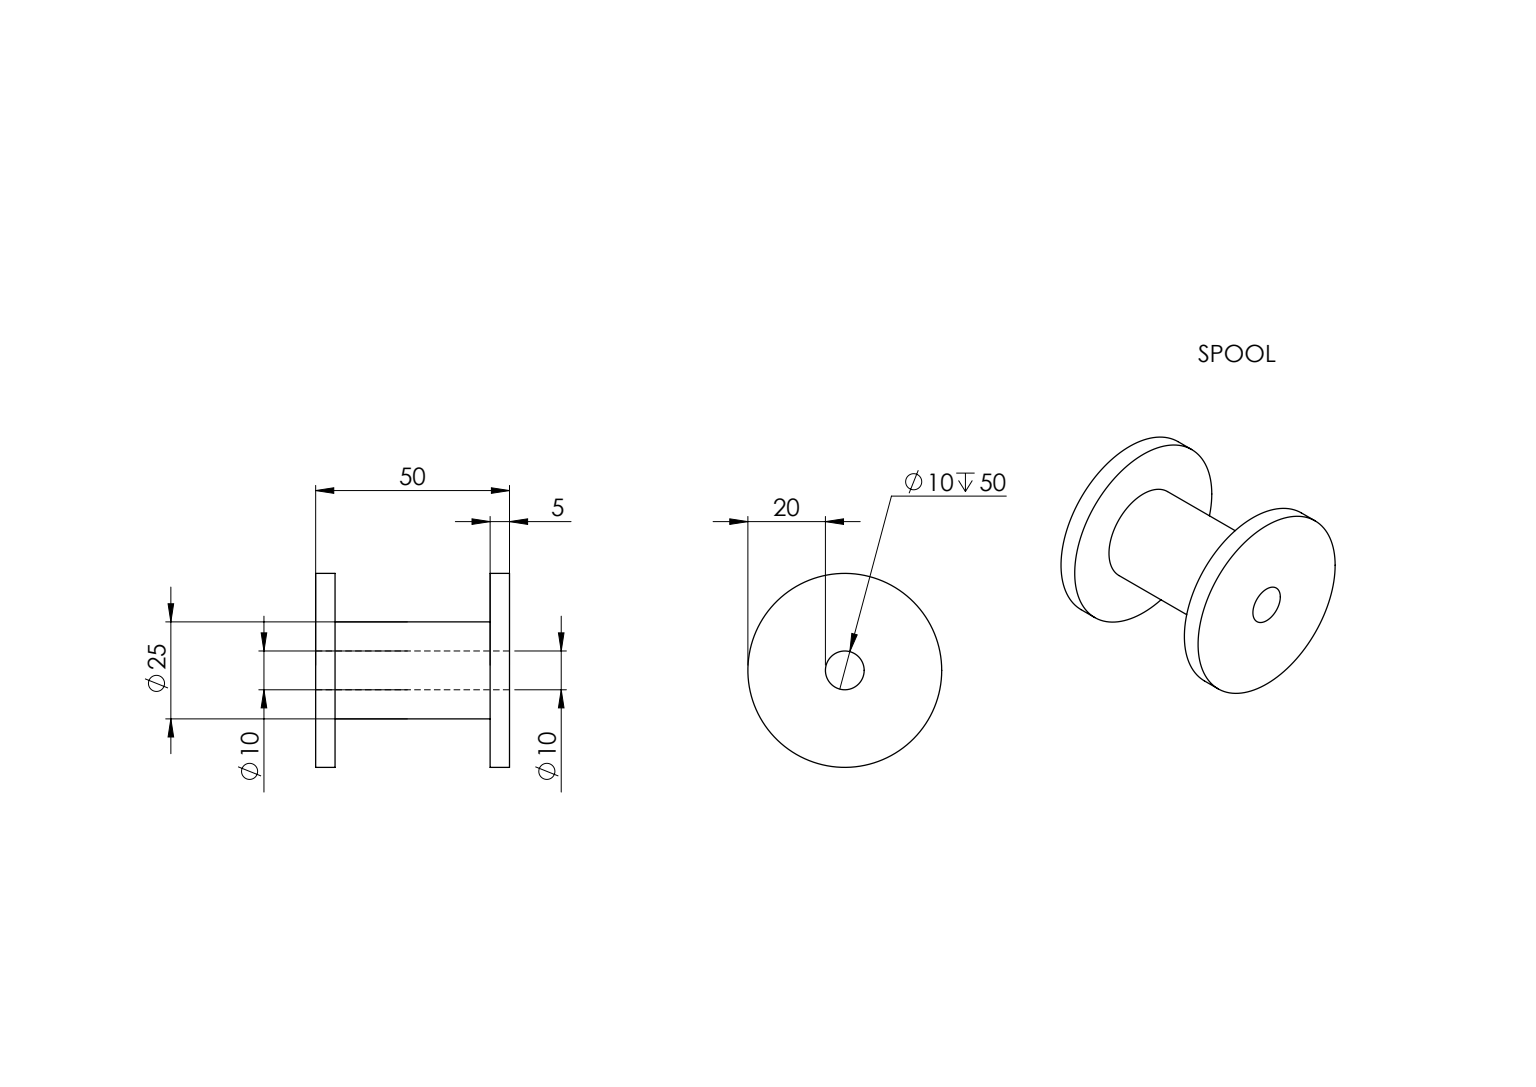
ISO-10303-21;
HEADER;
FILE_DESCRIPTION (('STEP AP214'),
    '1' );
FILE_NAME ('spool.step',
    '2026-10-27T08:02:39',
    ( '' ),
    ( '' ),
    'SwSTEP 2.0',
    'SolidWorks 2026',
    '' );
FILE_SCHEMA (( 'AUTOMOTIVE_DESIGN' ));
ENDSEC;

DATA;
#97=( NAMED_UNIT ( * ) SI_UNIT ( $, .STERADIAN. ) SOLID_ANGLE_UNIT ( ) );
#142=FACE_BOUND ( 'NONE', #771, .T. ) ;
#196=DIRECTION ( 'NONE',  ( 0.000000000000000000, 0.000000000000000000, 1.000000000000000000 ) ) ;
#212=CARTESIAN_POINT ( 'NONE',  ( 0.000000000000000000, 0.000000000000000000, 0.000000000000000000 ) ) ;
#226=DIRECTION ( 'NONE',  ( 1.000000000000000000, 0.000000000000000000, 0.000000000000000000 ) ) ;
#270=CARTESIAN_POINT ( 'NONE',  ( 25.00000000000000000, 0.000000000000000000, 0.000000000000000000 ) ) ;
#326=LINE ( 'NONE', #5141, #3967 ) ;
#355=LINE ( 'NONE', #8000, #10056 ) ;
#393=DIRECTION ( 'NONE',  ( 1.000000000000000000, 0.000000000000000000, 0.000000000000000000 ) ) ;
#459=CIRCLE ( 'NONE', #3072, 12.50000000000000000 ) ;
#620=AXIS2_PLACEMENT_3D ( 'NONE', #9988, #3488, #10977 ) ;
#625=CARTESIAN_POINT ( 'NONE',  ( -25.00000000000000000, 0.000000000000000000, 0.000000000000000000 ) ) ;
#642=CIRCLE ( 'NONE', #6043, 25.00000000000000000 ) ;
#671=FACE_BOUND ( 'NONE', #6645, .T. ) ;
#771=EDGE_LOOP ( 'NONE', ( #6888, #1800 ) ) ;
#957=DIRECTION ( 'NONE',  ( 1.000000000000000000, 0.000000000000000000, 0.000000000000000000 ) ) ;
#961=SURFACE_SIDE_STYLE ('',( #5858 ) ) ;
#980=EDGE_CURVE ( 'NONE', #1358, #1101, #4200, .T. ) ;
#1046=CARTESIAN_POINT ( 'NONE',  ( 20.00000000000000000, 3.061616997868383043E-15, 25.00000000000000000 ) ) ;
#1054=DIRECTION ( 'NONE',  ( 1.000000000000000000, 0.000000000000000000, 0.000000000000000000 ) ) ;
#1071=DIRECTION ( 'NONE',  ( 0.000000000000000000, 0.000000000000000000, 1.000000000000000000 ) ) ;
#1097=( NAMED_UNIT ( * ) PLANE_ANGLE_UNIT ( ) SI_UNIT ( $, .RADIAN. ) );
#1101=VERTEX_POINT ( 'NONE', #1046 ) ;
#1135=CARTESIAN_POINT ( 'NONE',  ( 25.00000000000000000, 0.000000000000000000, 0.000000000000000000 ) ) ;
#1142=FACE_OUTER_BOUND ( 'NONE', #11815, .T. ) ;
#1171=EDGE_CURVE ( 'NONE', #6684, #6331, #3612, .T. ) ;
#1213=FILL_AREA_STYLE ('',( #6917 ) ) ;
#1214=ORIENTED_EDGE ( 'NONE', *, *, #7345, .F. ) ;
#1267=ORIENTED_EDGE ( 'NONE', *, *, #10956, .F. ) ;
#1301=ORIENTED_EDGE ( 'NONE', *, *, #2405, .T. ) ;
#1314=FACE_OUTER_BOUND ( 'NONE', #4071, .T. ) ;
#1327=DIRECTION ( 'NONE',  ( 0.000000000000000000, 0.000000000000000000, -1.000000000000000000 ) ) ;
#1349=ORIENTED_EDGE ( 'NONE', *, *, #3855, .T. ) ;
#1358=VERTEX_POINT ( 'NONE', #5530 ) ;
#1364=VECTOR ( 'NONE', #12094, 1000.000000000000000 ) ;
#1402=CARTESIAN_POINT ( 'NONE',  ( 25.00000000000000000, 0.000000000000000000, 0.000000000000000000 ) ) ;
#1412=ORIENTED_EDGE ( 'NONE', *, *, #980, .F. ) ;
#1470=CARTESIAN_POINT ( 'NONE',  ( -20.00000000000000000, 0.000000000000000000, 0.000000000000000000 ) ) ;
#1514=DIRECTION ( 'NONE',  ( 0.000000000000000000, 0.000000000000000000, -1.000000000000000000 ) ) ;
#1630=DIRECTION ( 'NONE',  ( 1.000000000000000000, 0.000000000000000000, 0.000000000000000000 ) ) ;
#1657=VERTEX_POINT ( 'NONE', #3156 ) ;
#1730=DIRECTION ( 'NONE',  ( 0.000000000000000000, 0.000000000000000000, -1.000000000000000000 ) ) ;
#1731=EDGE_CURVE ( 'NONE', #6756, #7499, #326, .T. ) ;
#1747=VERTEX_POINT ( 'NONE', #10142 ) ;
#1777=CARTESIAN_POINT ( 'NONE',  ( -25.00000000000000000, 6.123233995736766282E-16, -5.000000000000000000 ) ) ;
#1793=ORIENTED_EDGE ( 'NONE', *, *, #9745, .F. ) ;
#1795=LINE ( 'NONE', #4305, #6226 ) ;
#1800=ORIENTED_EDGE ( 'NONE', *, *, #4057, .T. ) ;
#1916=EDGE_LOOP ( 'NONE', ( #11600, #6853 ) ) ;
#1917=( LENGTH_UNIT ( ) NAMED_UNIT ( * ) SI_UNIT ( .MILLI., .METRE. ) );
#1988=CARTESIAN_POINT ( 'NONE',  ( 25.00000000000000000, 0.000000000000000000, 0.000000000000000000 ) ) ;
#2080=MECHANICAL_DESIGN_GEOMETRIC_PRESENTATION_REPRESENTATION('',(#3887),#10866);
#2081=DIRECTION ( 'NONE',  ( 1.000000000000000000, -0.000000000000000000, -0.000000000000000000 ) ) ;
#2083=ORIENTED_EDGE ( 'NONE', *, *, #7345, .T. ) ;
#2120=ORIENTED_EDGE ( 'NONE', *, *, #9829, .F. ) ;
#2122=CARTESIAN_POINT ( 'NONE',  ( -19.99999999999999645, 0.000000000000000000, 12.50000000000000000 ) ) ;
#2150=SHAPE_DEFINITION_REPRESENTATION ( #8046, #7217 ) ;
#2179=ADVANCED_FACE ( 'NONE', ( #8194, #3447 ), #9138, .T. ) ;
#2211=ORIENTED_EDGE ( 'NONE', *, *, #8931, .F. ) ;
#2280=DIRECTION ( 'NONE',  ( 0.000000000000000000, 0.000000000000000000, -1.000000000000000000 ) ) ;
#2288=AXIS2_PLACEMENT_3D ( 'NONE', #7775, #11643, #9901 ) ;
#2395=( LENGTH_UNIT ( ) NAMED_UNIT ( * ) SI_UNIT ( .MILLI., .METRE. ) );
#2405=EDGE_CURVE ( 'NONE', #12064, #3807, #9823, .T. ) ;
#2527=DIRECTION ( 'NONE',  ( 1.000000000000000000, 0.000000000000000000, 0.000000000000000000 ) ) ;
#2578=ORIENTED_EDGE ( 'NONE', *, *, #10956, .T. ) ;
#2623=VERTEX_POINT ( 'NONE', #1777 ) ;
#2628=EDGE_CURVE ( 'NONE', #6331, #6684, #11193, .T. ) ;
#2679=EDGE_CURVE ( 'NONE', #6067, #9683, #10623, .T. ) ;
#2791=DIRECTION ( 'NONE',  ( -1.000000000000000000, -0.000000000000000000, -0.000000000000000000 ) ) ;
#2915=LINE ( 'NONE', #9730, #10436 ) ;
#2988=CLOSED_SHELL ( 'NONE', ( #5813, #5217, #3491, #8176, #5004, #4607, #4938, #11804, #6014, #11882, #2179, #7611 ) ) ;
#3002=FACE_OUTER_BOUND ( 'NONE', #7243, .T. ) ;
#3072=AXIS2_PLACEMENT_3D ( 'NONE', #4632, #4174, #7889 ) ;
#3078=ORIENTED_EDGE ( 'NONE', *, *, #11451, .T. ) ;
#3081=FACE_OUTER_BOUND ( 'NONE', #4296, .T. ) ;
#3090=CYLINDRICAL_SURFACE ( 'NONE', #11035, 5.000000000000000000 ) ;
#3156=CARTESIAN_POINT ( 'NONE',  ( -19.99999999999999645, 1.530808498934191521E-15, -12.50000000000000000 ) ) ;
#3211=ORIENTED_EDGE ( 'NONE', *, *, #12328, .F. ) ;
#3291=EDGE_LOOP ( 'NONE', ( #5014, #12285, #7753, #4819 ) ) ;
#3379=DIRECTION ( 'NONE',  ( 0.000000000000000000, 0.000000000000000000, -1.000000000000000000 ) ) ;
#3447=FACE_BOUND ( 'NONE', #1916, .T. ) ;
#3488=DIRECTION ( 'NONE',  ( 1.000000000000000000, 0.000000000000000000, 0.000000000000000000 ) ) ;
#3491=ADVANCED_FACE ( 'NONE', ( #1314 ), #3090, .F. ) ;
#3563=ORIENTED_EDGE ( 'NONE', *, *, #4057, .F. ) ;
#3574=CIRCLE ( 'NONE', #5763, 25.00000000000000000 ) ;
#3598=DIRECTION ( 'NONE',  ( 0.000000000000000000, 0.000000000000000000, -1.000000000000000000 ) ) ;
#3612=CIRCLE ( 'NONE', #6408, 25.00000000000000000 ) ;
#3635=CARTESIAN_POINT ( 'NONE',  ( 20.00000000000000000, 0.000000000000000000, 0.000000000000000000 ) ) ;
#3807=VERTEX_POINT ( 'NONE', #9382 ) ;
#3852=PRESENTATION_STYLE_ASSIGNMENT (( #5032 ) ) ;
#3855=EDGE_CURVE ( 'NONE', #9683, #6067, #459, .T. ) ;
#3859=COLOUR_RGB ( '',0.8941176470588234615, 0.8941176470588234615, 0.8941176470588234615 ) ;
#3869=CIRCLE ( 'NONE', #7870, 5.000000000000000000 ) ;
#3871=VERTEX_POINT ( 'NONE', #2122 ) ;
#3873=EDGE_CURVE ( 'NONE', #12064, #8607, #355, .T. ) ;
#3887=STYLED_ITEM('',(#12412),#4645);
#3905=UNCERTAINTY_MEASURE_WITH_UNIT (LENGTH_MEASURE( 1.000000000000000082E-05 ), #1917, 'distance_accuracy_value', 'NONE');
#3910=CARTESIAN_POINT ( 'NONE',  ( 25.00000000000000000, 6.123233995736766282E-16, -5.000000000000000000 ) ) ;
#3949=CARTESIAN_POINT ( 'NONE',  ( -19.99999999999999645, 0.000000000000000000, 0.000000000000000000 ) ) ;
#3956=FACE_OUTER_BOUND ( 'NONE', #11536, .T. ) ;
#3967=VECTOR ( 'NONE', #5024, 1000.000000000000000 ) ;
#3973=EDGE_CURVE ( 'NONE', #3871, #1657, #8067, .T. ) ;
#3980=ORIENTED_EDGE ( 'NONE', *, *, #9518, .T. ) ;
#4031=VECTOR ( 'NONE', #4905, 1000.000000000000000 ) ;
#4032=CIRCLE ( 'NONE', #9832, 25.00000000000000000 ) ;
#4035=DIRECTION ( 'NONE',  ( 0.000000000000000000, 0.000000000000000000, 1.000000000000000000 ) ) ;
#4038=CARTESIAN_POINT ( 'NONE',  ( 25.00000000000000000, 0.000000000000000000, 0.000000000000000000 ) ) ;
#4057=EDGE_CURVE ( 'NONE', #2623, #7499, #3869, .T. ) ;
#4071=EDGE_LOOP ( 'NONE', ( #3980, #9462, #7743, #9623 ) ) ;
#4083=DIRECTION ( 'NONE',  ( -1.000000000000000000, -0.000000000000000000, -0.000000000000000000 ) ) ;
#4093=AXIS2_PLACEMENT_3D ( 'NONE', #3635, #6273, #1514 ) ;
#4104=FACE_OUTER_BOUND ( 'NONE', #3291, .T. ) ;
#4111=ORIENTED_EDGE ( 'NONE', *, *, #9518, .F. ) ;
#4132=DIRECTION ( 'NONE',  ( -1.000000000000000000, -0.000000000000000000, -0.000000000000000000 ) ) ;
#4152=CARTESIAN_POINT ( 'NONE',  ( 25.00000000000000000, 0.000000000000000000, 0.000000000000000000 ) ) ;
#4174=DIRECTION ( 'NONE',  ( 1.000000000000000000, 0.000000000000000000, 0.000000000000000000 ) ) ;
#4200=CIRCLE ( 'NONE', #10797, 25.00000000000000000 ) ;
#4266=AXIS2_PLACEMENT_3D ( 'NONE', #4038, #393, #2280 ) ;
#4296=EDGE_LOOP ( 'NONE', ( #2120, #2578, #7552, #3563 ) ) ;
#4305=CARTESIAN_POINT ( 'NONE',  ( 25.00000000000000000, 1.530808498934191521E-15, -12.50000000000000000 ) ) ;
#4325=CARTESIAN_POINT ( 'NONE',  ( 20.00000000000000000, 1.530808498934191521E-15, -12.50000000000000000 ) ) ;
#4337=CYLINDRICAL_SURFACE ( 'NONE', #6991, 12.50000000000000000 ) ;
#4371=DIRECTION ( 'NONE',  ( 1.000000000000000000, -0.000000000000000000, -0.000000000000000000 ) ) ;
#4414=PLANE ( 'NONE',  #620 ) ;
#4421=DIRECTION ( 'NONE',  ( 1.000000000000000000, 0.000000000000000000, 0.000000000000000000 ) ) ;
#4445=DIRECTION ( 'NONE',  ( 0.000000000000000000, 0.000000000000000000, -1.000000000000000000 ) ) ;
#4452=VECTOR ( 'NONE', #7486, 1000.000000000000000 ) ;
#4480=ORIENTED_EDGE ( 'NONE', *, *, #2679, .F. ) ;
#4482=CARTESIAN_POINT ( 'NONE',  ( 20.00000000000000000, 0.000000000000000000, -25.00000000000000000 ) ) ;
#4516=LINE ( 'NONE', #6466, #8844 ) ;
#4552=ORIENTED_EDGE ( 'NONE', *, *, #1171, .T. ) ;
#4574=DIRECTION ( 'NONE',  ( -1.000000000000000000, -0.000000000000000000, -0.000000000000000000 ) ) ;
#4607=ADVANCED_FACE ( 'NONE', ( #6971, #7919 ), #10777, .T. ) ;
#4632=CARTESIAN_POINT ( 'NONE',  ( 20.00000000000000000, 0.000000000000000000, 0.000000000000000000 ) ) ;
#4645=MANIFOLD_SOLID_BREP ( 'Mirror2', #2988 ) ;
#4819=ORIENTED_EDGE ( 'NONE', *, *, #12183, .F. ) ;
#4905=DIRECTION ( 'NONE',  ( -1.000000000000000000, 0.000000000000000000, 0.000000000000000000 ) ) ;
#4938=ADVANCED_FACE ( 'NONE', ( #142, #3956 ), #7528, .F. ) ;
#5004=ADVANCED_FACE ( 'NONE', ( #1142 ), #7143, .T. ) ;
#5014=ORIENTED_EDGE ( 'NONE', *, *, #3855, .F. ) ;
#5024=DIRECTION ( 'NONE',  ( -1.000000000000000000, -0.000000000000000000, -0.000000000000000000 ) ) ;
#5031=AXIS2_PLACEMENT_3D ( 'NONE', #9171, #2527, #3598 ) ;
#5032=SURFACE_STYLE_USAGE ( .BOTH. , #961 ) ;
#5035=PRODUCT_CONTEXT ( 'NONE', #10489, 'mechanical' ) ;
#5084=EDGE_LOOP ( 'NONE', ( #9657, #11921, #6220, #1214 ) ) ;
#5141=CARTESIAN_POINT ( 'NONE',  ( 25.00000000000000000, 0.000000000000000000, 5.000000000000000000 ) ) ;
#5217=ADVANCED_FACE ( 'NONE', ( #9331 ), #11008, .T. ) ;
#5282=DIRECTION ( 'NONE',  ( -1.000000000000000000, 0.000000000000000000, 0.000000000000000000 ) ) ;
#5521=CARTESIAN_POINT ( 'NONE',  ( -25.00000000000000000, 0.000000000000000000, 5.000000000000000000 ) ) ;
#5530=CARTESIAN_POINT ( 'NONE',  ( 20.00000000000000000, 0.000000000000000000, -25.00000000000000000 ) ) ;
#5627=ORIENTED_EDGE ( 'NONE', *, *, #11451, .F. ) ;
#5679=ORIENTED_EDGE ( 'NONE', *, *, #3873, .T. ) ;
#5705=DIRECTION ( 'NONE',  ( 0.000000000000000000, 0.000000000000000000, -1.000000000000000000 ) ) ;
#5716=LINE ( 'NONE', #10587, #4031 ) ;
#5763=AXIS2_PLACEMENT_3D ( 'NONE', #10625, #6884, #10687 ) ;
#5782=( NAMED_UNIT ( * ) PLANE_ANGLE_UNIT ( ) SI_UNIT ( $, .RADIAN. ) );
#5813=ADVANCED_FACE ( 'NONE', ( #5881 ), #5988, .T. ) ;
#5858=SURFACE_STYLE_FILL_AREA ( #1213 ) ;
#5881=FACE_OUTER_BOUND ( 'NONE', #6089, .T. ) ;
#5893=CARTESIAN_POINT ( 'NONE',  ( 25.00000000000000000, 0.000000000000000000, 0.000000000000000000 ) ) ;
#5988=CYLINDRICAL_SURFACE ( 'NONE', #8423, 25.00000000000000000 ) ;
#6002=DIRECTION ( 'NONE',  ( 1.000000000000000000, 0.000000000000000000, 0.000000000000000000 ) ) ;
#6014=ADVANCED_FACE ( 'NONE', ( #6356, #671 ), #4414, .F. ) ;
#6043=AXIS2_PLACEMENT_3D ( 'NONE', #7149, #9104, #1327 ) ;
#6056=AXIS2_PLACEMENT_3D ( 'NONE', #212, #4035, #8864 ) ;
#6067=VERTEX_POINT ( 'NONE', #9250 ) ;
#6069=DIRECTION ( 'NONE',  ( 0.000000000000000000, 0.000000000000000000, -1.000000000000000000 ) ) ;
#6089=EDGE_LOOP ( 'NONE', ( #12305, #5679, #8687, #8501 ) ) ;
#6139=DIRECTION ( 'NONE',  ( 0.000000000000000000, 0.000000000000000000, 1.000000000000000000 ) ) ;
#6199=DIRECTION ( 'NONE',  ( 0.000000000000000000, 0.000000000000000000, -1.000000000000000000 ) ) ;
#6205=CARTESIAN_POINT ( 'NONE',  ( 25.00000000000000000, 0.000000000000000000, -25.00000000000000000 ) ) ;
#6220=ORIENTED_EDGE ( 'NONE', *, *, #2628, .F. ) ;
#6226=VECTOR ( 'NONE', #2791, 1000.000000000000000 ) ;
#6273=DIRECTION ( 'NONE',  ( 1.000000000000000000, 0.000000000000000000, 0.000000000000000000 ) ) ;
#6331=VERTEX_POINT ( 'NONE', #6205 ) ;
#6356=FACE_OUTER_BOUND ( 'NONE', #9351, .T. ) ;
#6374=DIRECTION ( 'NONE',  ( -0.000000000000000000, 0.000000000000000000, -1.000000000000000000 ) ) ;
#6408=AXIS2_PLACEMENT_3D ( 'NONE', #1402, #226, #7165 ) ;
#6413=CARTESIAN_POINT ( 'NONE',  ( 25.00000000000000000, 0.000000000000000000, 0.000000000000000000 ) ) ;
#6443=PRODUCT_DEFINITION_FORMATION_WITH_SPECIFIED_SOURCE ( 'ANY', '', #9134, .NOT_KNOWN. ) ;
#6456=CIRCLE ( 'NONE', #10238, 25.00000000000000000 ) ;
#6466=CARTESIAN_POINT ( 'NONE',  ( 25.00000000000000000, 6.123233995736766282E-16, -5.000000000000000000 ) ) ;
#6470=CYLINDRICAL_SURFACE ( 'NONE', #6783, 25.00000000000000000 ) ;
#6645=EDGE_LOOP ( 'NONE', ( #11341, #1349 ) ) ;
#6653=AXIS2_PLACEMENT_3D ( 'NONE', #5893, #9645, #1071 ) ;
#6684=VERTEX_POINT ( 'NONE', #7896 ) ;
#6756=VERTEX_POINT ( 'NONE', #11737 ) ;
#6783=AXIS2_PLACEMENT_3D ( 'NONE', #1470, #5282, #9107 ) ;
#6833=EDGE_LOOP ( 'NONE', ( #4111, #1267 ) ) ;
#6848=CIRCLE ( 'NONE', #7847, 5.000000000000000000 ) ;
#6853=ORIENTED_EDGE ( 'NONE', *, *, #10054, .F. ) ;
#6884=DIRECTION ( 'NONE',  ( 1.000000000000000000, -0.000000000000000000, -0.000000000000000000 ) ) ;
#6888=ORIENTED_EDGE ( 'NONE', *, *, #11947, .T. ) ;
#6917=FILL_AREA_STYLE_COLOUR ( '', #3859 ) ;
#6945=DIRECTION ( 'NONE',  ( 1.000000000000000000, 0.000000000000000000, 0.000000000000000000 ) ) ;
#6971=FACE_BOUND ( 'NONE', #6833, .T. ) ;
#6991=AXIS2_PLACEMENT_3D ( 'NONE', #4152, #7979, #7925 ) ;
#7056=CIRCLE ( 'NONE', #9063, 12.50000000000000000 ) ;
#7060=DIRECTION ( 'NONE',  ( -1.000000000000000000, 0.000000000000000000, 0.000000000000000000 ) ) ;
#7127=CARTESIAN_POINT ( 'NONE',  ( -25.00000000000000000, 0.000000000000000000, 0.000000000000000000 ) ) ;
#7143=CYLINDRICAL_SURFACE ( 'NONE', #9087, 12.50000000000000000 ) ;
#7149=CARTESIAN_POINT ( 'NONE',  ( 20.00000000000000000, 0.000000000000000000, 0.000000000000000000 ) ) ;
#7165=DIRECTION ( 'NONE',  ( 0.000000000000000000, 0.000000000000000000, -1.000000000000000000 ) ) ;
#7217=SHAPE_REPRESENTATION ( 'spool', ( #6056 ), #10046 ) ;
#7230=EDGE_CURVE ( 'NONE', #3807, #12064, #3574, .T. ) ;
#7243=EDGE_LOOP ( 'NONE', ( #3211, #9374, #2083, #11611 ) ) ;
#7292=ORIENTED_EDGE ( 'NONE', *, *, #3873, .F. ) ;
#7327=DIRECTION ( 'NONE',  ( 1.000000000000000000, 0.000000000000000000, -0.000000000000000000 ) ) ;
#7330=ORIENTED_EDGE ( 'NONE', *, *, #3973, .T. ) ;
#7345=EDGE_CURVE ( 'NONE', #1358, #6331, #8304, .T. ) ;
#7439=AXIS2_PLACEMENT_3D ( 'NONE', #7127, #6002, #9886 ) ;
#7486=DIRECTION ( 'NONE',  ( -1.000000000000000000, -0.000000000000000000, -0.000000000000000000 ) ) ;
#7499=VERTEX_POINT ( 'NONE', #5521 ) ;
#7528=PLANE ( 'NONE',  #2288 ) ;
#7552=ORIENTED_EDGE ( 'NONE', *, *, #1731, .T. ) ;
#7584=EDGE_LOOP ( 'NONE', ( #7292, #8128, #10911, #3078 ) ) ;
#7611=ADVANCED_FACE ( 'NONE', ( #8337 ), #6470, .T. ) ;
#7626=MECHANICAL_DESIGN_GEOMETRIC_PRESENTATION_REPRESENTATION('',(#7661),#8220);
#7661=STYLED_ITEM ( 'NONE', ( #3852 ), #10918 ) ;
#7688=CARTESIAN_POINT ( 'NONE',  ( -20.00000000000000000, 0.000000000000000000, 0.000000000000000000 ) ) ;
#7743=ORIENTED_EDGE ( 'NONE', *, *, #11947, .F. ) ;
#7753=ORIENTED_EDGE ( 'NONE', *, *, #10054, .T. ) ;
#7768=DIRECTION ( 'NONE',  ( 1.000000000000000000, -0.000000000000000000, -0.000000000000000000 ) ) ;
#7775=CARTESIAN_POINT ( 'NONE',  ( -25.00000000000000000, 0.000000000000000000, 0.000000000000000000 ) ) ;
#7786=DIRECTION ( 'NONE',  ( 0.000000000000000000, 0.000000000000000000, -1.000000000000000000 ) ) ;
#7847=AXIS2_PLACEMENT_3D ( 'NONE', #8789, #957, #7786 ) ;
#7870=AXIS2_PLACEMENT_3D ( 'NONE', #625, #1630, #4445 ) ;
#7889=DIRECTION ( 'NONE',  ( 0.000000000000000000, 0.000000000000000000, -1.000000000000000000 ) ) ;
#7896=CARTESIAN_POINT ( 'NONE',  ( 25.00000000000000000, 3.061616997868383043E-15, 25.00000000000000000 ) ) ;
#7917=( LENGTH_UNIT ( ) NAMED_UNIT ( * ) SI_UNIT ( .MILLI., .METRE. ) );
#7919=FACE_OUTER_BOUND ( 'NONE', #9077, .T. ) ;
#7925=DIRECTION ( 'NONE',  ( 0.000000000000000000, 0.000000000000000000, 1.000000000000000000 ) ) ;
#7958=CARTESIAN_POINT ( 'NONE',  ( -25.00000000000000000, 0.000000000000000000, 0.000000000000000000 ) ) ;
#7979=DIRECTION ( 'NONE',  ( -1.000000000000000000, -0.000000000000000000, -0.000000000000000000 ) ) ;
#8000=CARTESIAN_POINT ( 'NONE',  ( -20.00000000000000000, 3.061616997868383043E-15, -25.00000000000000000 ) ) ;
#8019=AXIS2_PLACEMENT_3D ( 'NONE', #7688, #10611, #8554 ) ;
#8046=PRODUCT_DEFINITION_SHAPE ( 'NONE', 'NONE',  #8872 ) ;
#8067=CIRCLE ( 'NONE', #11640, 12.50000000000000000 ) ;
#8128=ORIENTED_EDGE ( 'NONE', *, *, #7230, .F. ) ;
#8138=CARTESIAN_POINT ( 'NONE',  ( -20.00000000000000000, 0.000000000000000000, 0.000000000000000000 ) ) ;
#8176=ADVANCED_FACE ( 'NONE', ( #4104 ), #4337, .T. ) ;
#8194=FACE_OUTER_BOUND ( 'NONE', #9023, .T. ) ;
#8220=( GEOMETRIC_REPRESENTATION_CONTEXT ( 3 ) GLOBAL_UNCERTAINTY_ASSIGNED_CONTEXT ( ( #3905 ) ) GLOBAL_UNIT_ASSIGNED_CONTEXT ( ( #1917, #5782, #97 ) ) REPRESENTATION_CONTEXT ( 'NONE', 'WORKASPACE' ) );
#8304=LINE ( 'NONE', #4482, #1364 ) ;
#8337=FACE_OUTER_BOUND ( 'NONE', #7584, .T. ) ;
#8423=AXIS2_PLACEMENT_3D ( 'NONE', #8934, #7060, #11786 ) ;
#8501=ORIENTED_EDGE ( 'NONE', *, *, #9636, .F. ) ;
#8554=DIRECTION ( 'NONE',  ( 0.000000000000000000, 0.000000000000000000, -1.000000000000000000 ) ) ;
#8607=VERTEX_POINT ( 'NONE', #10317 ) ;
#8687=ORIENTED_EDGE ( 'NONE', *, *, #10071, .T. ) ;
#8789=CARTESIAN_POINT ( 'NONE',  ( 25.00000000000000000, 0.000000000000000000, 0.000000000000000000 ) ) ;
#8792=DIRECTION ( 'NONE',  ( 1.000000000000000000, 0.000000000000000000, 0.000000000000000000 ) ) ;
#8815=APPLICATION_CONTEXT ( 'automotive_design' ) ;
#8844=VECTOR ( 'NONE', #4574, 1000.000000000000000 ) ;
#8864=DIRECTION ( 'NONE',  ( 1.000000000000000000, 0.000000000000000000, 0.000000000000000000 ) ) ;
#8872=PRODUCT_DEFINITION ( 'UNKNOWN', '', #6443, #11644 ) ;
#8931=EDGE_CURVE ( 'NONE', #9683, #1657, #1795, .T. ) ;
#8934=CARTESIAN_POINT ( 'NONE',  ( -20.00000000000000000, 0.000000000000000000, 0.000000000000000000 ) ) ;
#9006=CARTESIAN_POINT ( 'NONE',  ( 20.00000000000000000, 0.000000000000000000, 0.000000000000000000 ) ) ;
#9010=AXIS2_PLACEMENT_3D ( 'NONE', #8138, #7327, #6374 ) ;
#9023=EDGE_LOOP ( 'NONE', ( #9075, #1301 ) ) ;
#9063=AXIS2_PLACEMENT_3D ( 'NONE', #3949, #7768, #11558 ) ;
#9075=ORIENTED_EDGE ( 'NONE', *, *, #7230, .T. ) ;
#9077=EDGE_LOOP ( 'NONE', ( #9925, #4552 ) ) ;
#9087=AXIS2_PLACEMENT_3D ( 'NONE', #270, #4083, #6139 ) ;
#9104=DIRECTION ( 'NONE',  ( 1.000000000000000000, 0.000000000000000000, 0.000000000000000000 ) ) ;
#9107=DIRECTION ( 'NONE',  ( 0.000000000000000000, 0.000000000000000000, 1.000000000000000000 ) ) ;
#9134=PRODUCT ( 'spool', 'spool', '', ( #5035 ) ) ;
#9138=PLANE ( 'NONE',  #9010 ) ;
#9160=( NAMED_UNIT ( * ) PLANE_ANGLE_UNIT ( ) SI_UNIT ( $, .RADIAN. ) );
#9171=CARTESIAN_POINT ( 'NONE',  ( 20.00000000000000000, 0.000000000000000000, 0.000000000000000000 ) ) ;
#9179=AXIS2_PLACEMENT_3D ( 'NONE', #1988, #1054, #10424 ) ;
#9250=CARTESIAN_POINT ( 'NONE',  ( 20.00000000000000000, 0.000000000000000000, 12.50000000000000000 ) ) ;
#9312=CARTESIAN_POINT ( 'NONE',  ( 20.00000000000000000, 0.000000000000000000, 0.000000000000000000 ) ) ;
#9331=FACE_OUTER_BOUND ( 'NONE', #5084, .T. ) ;
#9351=EDGE_LOOP ( 'NONE', ( #1412, #1793 ) ) ;
#9374=ORIENTED_EDGE ( 'NONE', *, *, #9745, .T. ) ;
#9382=CARTESIAN_POINT ( 'NONE',  ( -20.00000000000000000, 0.000000000000000000, 25.00000000000000000 ) ) ;
#9462=ORIENTED_EDGE ( 'NONE', *, *, #9829, .T. ) ;
#9518=EDGE_CURVE ( 'NONE', #6756, #9537, #6848, .T. ) ;
#9537=VERTEX_POINT ( 'NONE', #3910 ) ;
#9539=( NAMED_UNIT ( * ) SI_UNIT ( $, .STERADIAN. ) SOLID_ANGLE_UNIT ( ) );
#9623=ORIENTED_EDGE ( 'NONE', *, *, #1731, .F. ) ;
#9636=EDGE_CURVE ( 'NONE', #3807, #1747, #5716, .T. ) ;
#9645=DIRECTION ( 'NONE',  ( -1.000000000000000000, -0.000000000000000000, -0.000000000000000000 ) ) ;
#9657=ORIENTED_EDGE ( 'NONE', *, *, #980, .T. ) ;
#9673=SHAPE_REPRESENTATION_RELATIONSHIP ( 'NONE' , 'NONE' ,  #7217, #10918 ) ;
#9683=VERTEX_POINT ( 'NONE', #4325 ) ;
#9730=CARTESIAN_POINT ( 'NONE',  ( 20.00000000000000000, 3.061616997868383043E-15, 25.00000000000000000 ) ) ;
#9745=EDGE_CURVE ( 'NONE', #1101, #1358, #642, .T. ) ;
#9759=CYLINDRICAL_SURFACE ( 'NONE', #6653, 5.000000000000000000 ) ;
#9823=CIRCLE ( 'NONE', #8019, 25.00000000000000000 ) ;
#9829=EDGE_CURVE ( 'NONE', #9537, #2623, #4516, .T. ) ;
#9832=AXIS2_PLACEMENT_3D ( 'NONE', #7958, #4371, #3379 ) ;
#9849=CIRCLE ( 'NONE', #7439, 5.000000000000000000 ) ;
#9886=DIRECTION ( 'NONE',  ( 0.000000000000000000, 0.000000000000000000, -1.000000000000000000 ) ) ;
#9901=DIRECTION ( 'NONE',  ( 0.000000000000000000, 0.000000000000000000, -1.000000000000000000 ) ) ;
#9925=ORIENTED_EDGE ( 'NONE', *, *, #2628, .T. ) ;
#9988=CARTESIAN_POINT ( 'NONE',  ( 20.00000000000000000, 0.000000000000000000, 0.000000000000000000 ) ) ;
#10046=( GEOMETRIC_REPRESENTATION_CONTEXT ( 3 ) GLOBAL_UNCERTAINTY_ASSIGNED_CONTEXT ( ( #12262 ) ) GLOBAL_UNIT_ASSIGNED_CONTEXT ( ( #7917, #1097, #9539 ) ) REPRESENTATION_CONTEXT ( 'NONE', 'WORKASPACE' ) );
#10054=EDGE_CURVE ( 'NONE', #1657, #3871, #7056, .T. ) ;
#10056=VECTOR ( 'NONE', #11682, 1000.000000000000000 ) ;
#10071=EDGE_CURVE ( 'NONE', #8607, #1747, #6456, .T. ) ;
#10082=DIRECTION ( 'NONE',  ( 1.000000000000000000, -0.000000000000000000, -0.000000000000000000 ) ) ;
#10142=CARTESIAN_POINT ( 'NONE',  ( -25.00000000000000000, 0.000000000000000000, 25.00000000000000000 ) ) ;
#10238=AXIS2_PLACEMENT_3D ( 'NONE', #10647, #2081, #5705 ) ;
#10285=CARTESIAN_POINT ( 'NONE',  ( 25.00000000000000000, 0.000000000000000000, 12.50000000000000000 ) ) ;
#10289=ORIENTED_EDGE ( 'NONE', *, *, #10071, .F. ) ;
#10317=CARTESIAN_POINT ( 'NONE',  ( -25.00000000000000000, 3.061616997868383043E-15, -25.00000000000000000 ) ) ;
#10405=AXIS2_PLACEMENT_3D ( 'NONE', #6413, #11279, #12139 ) ;
#10424=DIRECTION ( 'NONE',  ( 0.000000000000000000, 0.000000000000000000, -1.000000000000000000 ) ) ;
#10427=AXIS2_PLACEMENT_3D ( 'NONE', #9006, #6945, #6069 ) ;
#10436=VECTOR ( 'NONE', #8792, 1000.000000000000000 ) ;
#10489=APPLICATION_CONTEXT ( 'automotive_design' ) ;
#10587=CARTESIAN_POINT ( 'NONE',  ( -20.00000000000000000, 0.000000000000000000, 25.00000000000000000 ) ) ;
#10611=DIRECTION ( 'NONE',  ( 1.000000000000000000, -0.000000000000000000, -0.000000000000000000 ) ) ;
#10623=CIRCLE ( 'NONE', #5031, 12.50000000000000000 ) ;
#10625=CARTESIAN_POINT ( 'NONE',  ( -20.00000000000000000, 0.000000000000000000, 0.000000000000000000 ) ) ;
#10647=CARTESIAN_POINT ( 'NONE',  ( -25.00000000000000000, 0.000000000000000000, 0.000000000000000000 ) ) ;
#10687=DIRECTION ( 'NONE',  ( 0.000000000000000000, 0.000000000000000000, -1.000000000000000000 ) ) ;
#10777=PLANE ( 'NONE',  #4266 ) ;
#10797=AXIS2_PLACEMENT_3D ( 'NONE', #9312, #4421, #1730 ) ;
#10866=( GEOMETRIC_REPRESENTATION_CONTEXT ( 3 ) GLOBAL_UNCERTAINTY_ASSIGNED_CONTEXT ( ( #11144 ) ) GLOBAL_UNIT_ASSIGNED_CONTEXT ( ( #2395, #9160, #12019 ) ) REPRESENTATION_CONTEXT ( 'NONE', 'WORKASPACE' ) );
#10910=CARTESIAN_POINT ( 'NONE',  ( -20.00000000000000000, 3.061616997868383043E-15, -25.00000000000000000 ) ) ;
#10911=ORIENTED_EDGE ( 'NONE', *, *, #9636, .T. ) ;
#10918=ADVANCED_BREP_SHAPE_REPRESENTATION ( '', ( #4645, #6056 ), #10046 ) ;
#10956=EDGE_CURVE ( 'NONE', #9537, #6756, #12350, .T. ) ;
#10977=DIRECTION ( 'NONE',  ( 0.000000000000000000, 0.000000000000000000, -1.000000000000000000 ) ) ;
#11008=CYLINDRICAL_SURFACE ( 'NONE', #4093, 25.00000000000000000 ) ;
#11035=AXIS2_PLACEMENT_3D ( 'NONE', #1135, #4132, #196 ) ;
#11123=CARTESIAN_POINT ( 'NONE',  ( -19.99999999999999645, 0.000000000000000000, 0.000000000000000000 ) ) ;
#11144=UNCERTAINTY_MEASURE_WITH_UNIT (LENGTH_MEASURE( 1.000000000000000082E-05 ), #2395, 'distance_accuracy_value', 'NONE');
#11193=CIRCLE ( 'NONE', #10405, 25.00000000000000000 ) ;
#11279=DIRECTION ( 'NONE',  ( 1.000000000000000000, 0.000000000000000000, 0.000000000000000000 ) ) ;
#11341=ORIENTED_EDGE ( 'NONE', *, *, #2679, .T. ) ;
#11342=ORIENTED_EDGE ( 'NONE', *, *, #12183, .T. ) ;
#11451=EDGE_CURVE ( 'NONE', #1747, #8607, #4032, .T. ) ;
#11536=EDGE_LOOP ( 'NONE', ( #5627, #10289 ) ) ;
#11558=DIRECTION ( 'NONE',  ( 0.000000000000000000, 0.000000000000000000, -1.000000000000000000 ) ) ;
#11600=ORIENTED_EDGE ( 'NONE', *, *, #3973, .F. ) ;
#11611=ORIENTED_EDGE ( 'NONE', *, *, #1171, .F. ) ;
#11640=AXIS2_PLACEMENT_3D ( 'NONE', #11123, #10082, #6199 ) ;
#11643=DIRECTION ( 'NONE',  ( 1.000000000000000000, 0.000000000000000000, 0.000000000000000000 ) ) ;
#11644=PRODUCT_DEFINITION_CONTEXT ( 'detailed design', #8815, 'design' ) ;
#11682=DIRECTION ( 'NONE',  ( -1.000000000000000000, 0.000000000000000000, 0.000000000000000000 ) ) ;
#11733=CYLINDRICAL_SURFACE ( 'NONE', #10427, 25.00000000000000000 ) ;
#11737=CARTESIAN_POINT ( 'NONE',  ( 25.00000000000000000, 0.000000000000000000, 5.000000000000000000 ) ) ;
#11786=DIRECTION ( 'NONE',  ( 0.000000000000000000, 0.000000000000000000, 1.000000000000000000 ) ) ;
#11804=ADVANCED_FACE ( 'NONE', ( #3081 ), #9759, .F. ) ;
#11815=EDGE_LOOP ( 'NONE', ( #2211, #4480, #11342, #7330 ) ) ;
#11882=ADVANCED_FACE ( 'NONE', ( #3002 ), #11733, .T. ) ;
#11921=ORIENTED_EDGE ( 'NONE', *, *, #12328, .T. ) ;
#11947=EDGE_CURVE ( 'NONE', #7499, #2623, #9849, .T. ) ;
#12019=( NAMED_UNIT ( * ) SI_UNIT ( $, .STERADIAN. ) SOLID_ANGLE_UNIT ( ) );
#12064=VERTEX_POINT ( 'NONE', #10910 ) ;
#12094=DIRECTION ( 'NONE',  ( 1.000000000000000000, 0.000000000000000000, 0.000000000000000000 ) ) ;
#12139=DIRECTION ( 'NONE',  ( 0.000000000000000000, 0.000000000000000000, -1.000000000000000000 ) ) ;
#12183=EDGE_CURVE ( 'NONE', #6067, #3871, #12329, .T. ) ;
#12262=UNCERTAINTY_MEASURE_WITH_UNIT (LENGTH_MEASURE( 1.000000000000000082E-05 ), #7917, 'distance_accuracy_value', 'NONE');
#12285=ORIENTED_EDGE ( 'NONE', *, *, #8931, .T. ) ;
#12305=ORIENTED_EDGE ( 'NONE', *, *, #2405, .F. ) ;
#12328=EDGE_CURVE ( 'NONE', #1101, #6684, #2915, .T. ) ;
#12329=LINE ( 'NONE', #10285, #4452 ) ;
#12350=CIRCLE ( 'NONE', #9179, 5.000000000000000000 ) ;
#12406=COLOUR_RGB('Off White',0.89,0.88,0.83);
#12407=FILL_AREA_STYLE_COLOUR('',#12406);
#12408=FILL_AREA_STYLE('',(#12407));
#12409=SURFACE_STYLE_FILL_AREA(#12408);
#12410=SURFACE_SIDE_STYLE('',(#12409));
#12411=SURFACE_STYLE_USAGE(.BOTH.,#12410);
#12412=PRESENTATION_STYLE_ASSIGNMENT((#12411));
ENDSEC;
END-ISO-10303-21;
